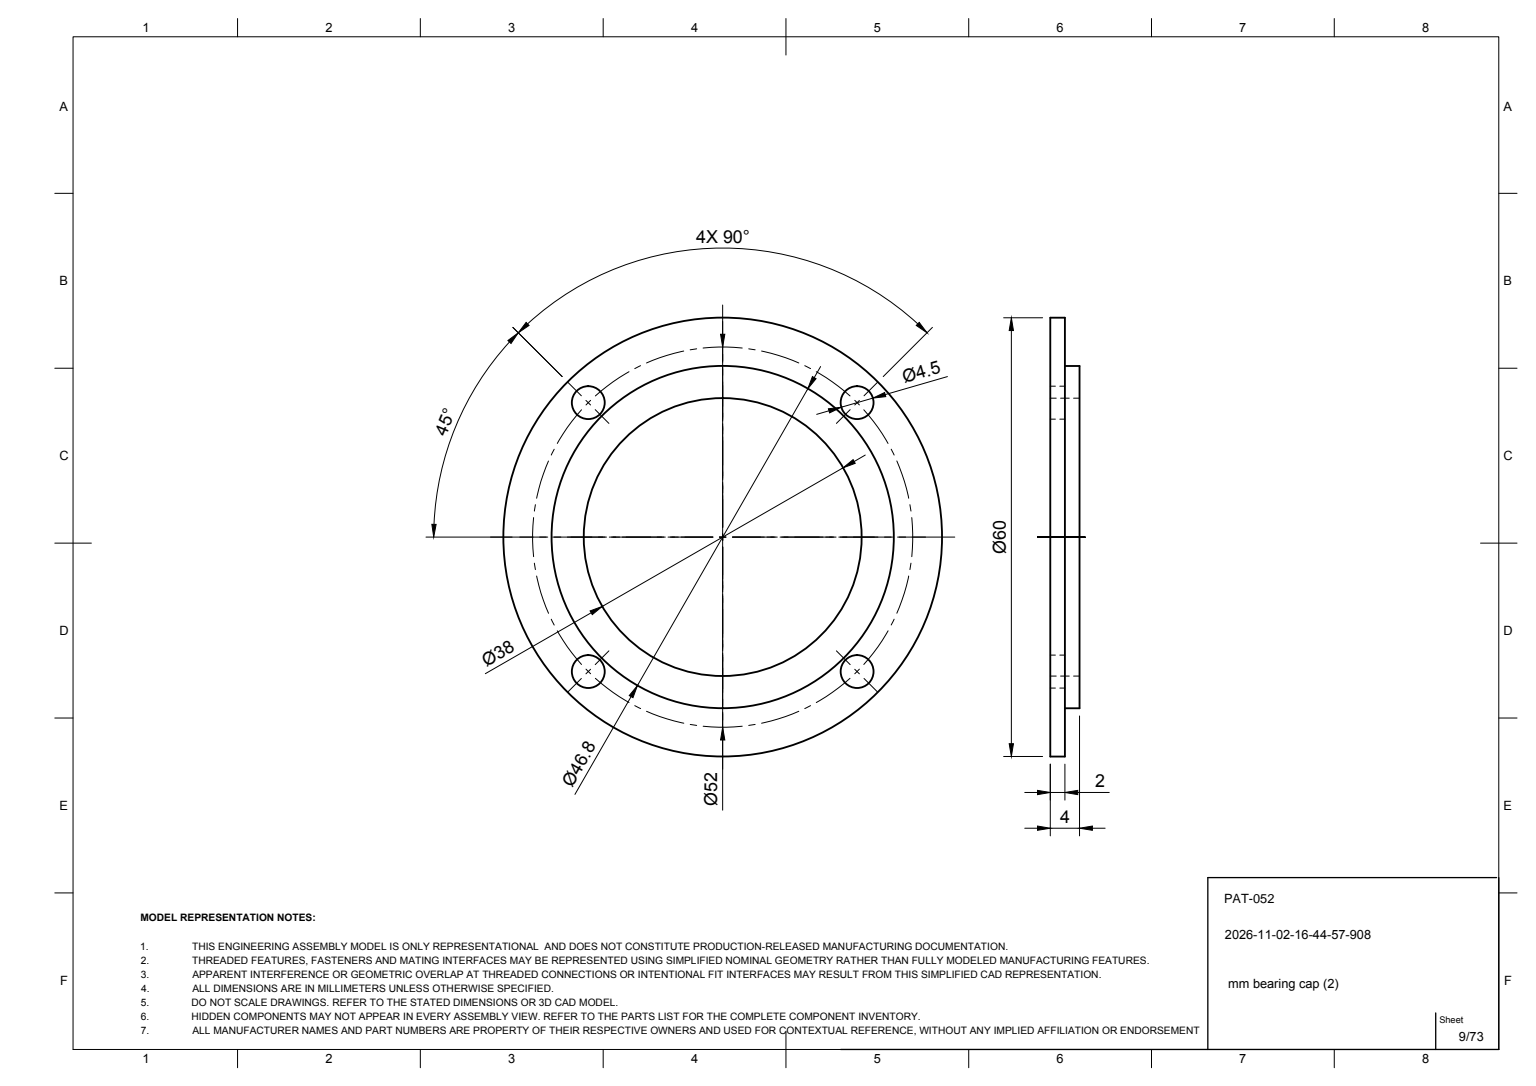
ISO-10303-21;
HEADER;
/* Generated by software containing ST-Developer
 * from STEP Tools, Inc. (www.steptools.com) 
 */

FILE_DESCRIPTION(
/* description */ ('Hand-crank gear train demonstrator'),
/* implementation_level */ '2;1');

FILE_NAME(
/* name */ 'mm bearing cap (2).step',
/* time_stamp */ '2026-10-28T03:22:13-07:00',
/* author */ (''),
/* organization */ (''),
/* preprocessor_version */ 'ST-DEVELOPER v20.2',
/* originating_system */ 'Autodesk Translation Framework v15.17.0.0',
/* authorisation */ '');

FILE_SCHEMA (('AUTOMOTIVE_DESIGN { 1 0 10303 214 3 1 1 }'));
ENDSEC;

DATA;
#10=MECHANICAL_DESIGN_GEOMETRIC_PRESENTATION_REPRESENTATION('',(#1193),#62758);
#1065=SHAPE_REPRESENTATION_RELATIONSHIP('SRR','None',#63037,#1129);
#1129=ADVANCED_BREP_SHAPE_REPRESENTATION('',(#1272),#62691);
#1193=STYLED_ITEM('',(#63462),#1272);
#1272=MANIFOLD_SOLID_BREP('Body1',#16373);
#1420=FACE_BOUND('',#3205,.T.);
#1421=FACE_BOUND('',#3209,.T.);
#1422=FACE_BOUND('',#3210,.T.);
#1423=FACE_BOUND('',#3211,.T.);
#1424=FACE_BOUND('',#3212,.T.);
#1425=FACE_BOUND('',#3213,.T.);
#1426=FACE_BOUND('',#3215,.T.);
#1427=FACE_BOUND('',#3216,.T.);
#1428=FACE_BOUND('',#3217,.T.);
#1429=FACE_BOUND('',#3218,.T.);
#1430=FACE_BOUND('',#3219,.T.);
#1653=PLANE('',#17326);
#1654=PLANE('',#17333);
#1655=PLANE('',#17334);
#2185=FACE_OUTER_BOUND('',#3199,.T.);
#2186=FACE_OUTER_BOUND('',#3200,.T.);
#2187=FACE_OUTER_BOUND('',#3201,.T.);
#2188=FACE_OUTER_BOUND('',#3202,.T.);
#2189=FACE_OUTER_BOUND('',#3203,.T.);
#2190=FACE_OUTER_BOUND('',#3204,.T.);
#2191=FACE_OUTER_BOUND('',#3206,.T.);
#2192=FACE_OUTER_BOUND('',#3207,.T.);
#2193=FACE_OUTER_BOUND('',#3208,.T.);
#2194=FACE_OUTER_BOUND('',#3214,.T.);
#3199=EDGE_LOOP('',(#11147,#11148,#11149,#11150));
#3200=EDGE_LOOP('',(#11151,#11152,#11153,#11154));
#3201=EDGE_LOOP('',(#11155,#11156,#11157,#11158));
#3202=EDGE_LOOP('',(#11159,#11160,#11161,#11162));
#3203=EDGE_LOOP('',(#11163,#11164,#11165,#11166));
#3204=EDGE_LOOP('',(#11167));
#3205=EDGE_LOOP('',(#11168));
#3206=EDGE_LOOP('',(#11169,#11170,#11171,#11172));
#3207=EDGE_LOOP('',(#11173,#11174,#11175,#11176));
#3208=EDGE_LOOP('',(#11177));
#3209=EDGE_LOOP('',(#11178));
#3210=EDGE_LOOP('',(#11179));
#3211=EDGE_LOOP('',(#11180));
#3212=EDGE_LOOP('',(#11181));
#3213=EDGE_LOOP('',(#11182));
#3214=EDGE_LOOP('',(#11183));
#3215=EDGE_LOOP('',(#11184));
#3216=EDGE_LOOP('',(#11185));
#3217=EDGE_LOOP('',(#11186));
#3218=EDGE_LOOP('',(#11187));
#3219=EDGE_LOOP('',(#11188));
#4358=LINE('',#23642,#5490);
#4359=LINE('',#23648,#5491);
#4360=LINE('',#23654,#5492);
#4361=LINE('',#23660,#5493);
#4362=LINE('',#23666,#5494);
#4363=LINE('',#23673,#5495);
#4364=LINE('',#23679,#5496);
#5490=VECTOR('',#19213,0.225);
#5491=VECTOR('',#19220,0.225);
#5492=VECTOR('',#19227,0.225000000000001);
#5493=VECTOR('',#19234,0.225000000000001);
#5494=VECTOR('',#19241,2.34);
#5495=VECTOR('',#19250,1.9);
#5496=VECTOR('',#19257,3.);
#6634=CIRCLE('',#17312,0.225);
#6635=CIRCLE('',#17313,0.225);
#6636=CIRCLE('',#17315,0.225);
#6637=CIRCLE('',#17316,0.225);
#6638=CIRCLE('',#17318,0.225000000000001);
#6639=CIRCLE('',#17319,0.225000000000001);
#6640=CIRCLE('',#17321,0.225000000000001);
#6641=CIRCLE('',#17322,0.225000000000001);
#6642=CIRCLE('',#17324,2.34);
#6643=CIRCLE('',#17325,2.34);
#6644=CIRCLE('',#17327,1.9);
#6645=CIRCLE('',#17329,1.9);
#6646=CIRCLE('',#17331,3.);
#6647=CIRCLE('',#17332,3.);
#7316=VERTEX_POINT('',#23639);
#7317=VERTEX_POINT('',#23641);
#7318=VERTEX_POINT('',#23645);
#7319=VERTEX_POINT('',#23647);
#7320=VERTEX_POINT('',#23651);
#7321=VERTEX_POINT('',#23653);
#7322=VERTEX_POINT('',#23657);
#7323=VERTEX_POINT('',#23659);
#7324=VERTEX_POINT('',#23663);
#7325=VERTEX_POINT('',#23665);
#7326=VERTEX_POINT('',#23669);
#7327=VERTEX_POINT('',#23672);
#7328=VERTEX_POINT('',#23676);
#7329=VERTEX_POINT('',#23678);
#8825=EDGE_CURVE('',#7316,#7316,#6634,.T.);
#8826=EDGE_CURVE('',#7316,#7317,#4358,.T.);
#8827=EDGE_CURVE('',#7317,#7317,#6635,.T.);
#8828=EDGE_CURVE('',#7318,#7318,#6636,.T.);
#8829=EDGE_CURVE('',#7318,#7319,#4359,.T.);
#8830=EDGE_CURVE('',#7319,#7319,#6637,.T.);
#8831=EDGE_CURVE('',#7320,#7320,#6638,.T.);
#8832=EDGE_CURVE('',#7320,#7321,#4360,.T.);
#8833=EDGE_CURVE('',#7321,#7321,#6639,.T.);
#8834=EDGE_CURVE('',#7322,#7322,#6640,.T.);
#8835=EDGE_CURVE('',#7322,#7323,#4361,.T.);
#8836=EDGE_CURVE('',#7323,#7323,#6641,.T.);
#8837=EDGE_CURVE('',#7324,#7324,#6642,.T.);
#8838=EDGE_CURVE('',#7324,#7325,#4362,.T.);
#8839=EDGE_CURVE('',#7325,#7325,#6643,.T.);
#8840=EDGE_CURVE('',#7326,#7326,#6644,.T.);
#8841=EDGE_CURVE('',#7326,#7327,#4363,.T.);
#8842=EDGE_CURVE('',#7327,#7327,#6645,.T.);
#8843=EDGE_CURVE('',#7328,#7328,#6646,.T.);
#8844=EDGE_CURVE('',#7328,#7329,#4364,.T.);
#8845=EDGE_CURVE('',#7329,#7329,#6647,.T.);
#11147=ORIENTED_EDGE('',*,*,#8825,.F.);
#11148=ORIENTED_EDGE('',*,*,#8826,.T.);
#11149=ORIENTED_EDGE('',*,*,#8827,.F.);
#11150=ORIENTED_EDGE('',*,*,#8826,.F.);
#11151=ORIENTED_EDGE('',*,*,#8828,.F.);
#11152=ORIENTED_EDGE('',*,*,#8829,.T.);
#11153=ORIENTED_EDGE('',*,*,#8830,.F.);
#11154=ORIENTED_EDGE('',*,*,#8829,.F.);
#11155=ORIENTED_EDGE('',*,*,#8831,.F.);
#11156=ORIENTED_EDGE('',*,*,#8832,.T.);
#11157=ORIENTED_EDGE('',*,*,#8833,.F.);
#11158=ORIENTED_EDGE('',*,*,#8832,.F.);
#11159=ORIENTED_EDGE('',*,*,#8834,.F.);
#11160=ORIENTED_EDGE('',*,*,#8835,.T.);
#11161=ORIENTED_EDGE('',*,*,#8836,.F.);
#11162=ORIENTED_EDGE('',*,*,#8835,.F.);
#11163=ORIENTED_EDGE('',*,*,#8837,.F.);
#11164=ORIENTED_EDGE('',*,*,#8838,.T.);
#11165=ORIENTED_EDGE('',*,*,#8839,.F.);
#11166=ORIENTED_EDGE('',*,*,#8838,.F.);
#11167=ORIENTED_EDGE('',*,*,#8837,.T.);
#11168=ORIENTED_EDGE('',*,*,#8840,.T.);
#11169=ORIENTED_EDGE('',*,*,#8840,.F.);
#11170=ORIENTED_EDGE('',*,*,#8841,.T.);
#11171=ORIENTED_EDGE('',*,*,#8842,.T.);
#11172=ORIENTED_EDGE('',*,*,#8841,.F.);
#11173=ORIENTED_EDGE('',*,*,#8843,.F.);
#11174=ORIENTED_EDGE('',*,*,#8844,.T.);
#11175=ORIENTED_EDGE('',*,*,#8845,.T.);
#11176=ORIENTED_EDGE('',*,*,#8844,.F.);
#11177=ORIENTED_EDGE('',*,*,#8843,.T.);
#11178=ORIENTED_EDGE('',*,*,#8839,.T.);
#11179=ORIENTED_EDGE('',*,*,#8836,.T.);
#11180=ORIENTED_EDGE('',*,*,#8833,.T.);
#11181=ORIENTED_EDGE('',*,*,#8830,.T.);
#11182=ORIENTED_EDGE('',*,*,#8827,.T.);
#11183=ORIENTED_EDGE('',*,*,#8845,.F.);
#11184=ORIENTED_EDGE('',*,*,#8842,.F.);
#11185=ORIENTED_EDGE('',*,*,#8834,.T.);
#11186=ORIENTED_EDGE('',*,*,#8831,.T.);
#11187=ORIENTED_EDGE('',*,*,#8828,.T.);
#11188=ORIENTED_EDGE('',*,*,#8825,.T.);
#15209=CYLINDRICAL_SURFACE('',#17311,0.225);
#15210=CYLINDRICAL_SURFACE('',#17314,0.225);
#15211=CYLINDRICAL_SURFACE('',#17317,0.225000000000001);
#15212=CYLINDRICAL_SURFACE('',#17320,0.225000000000001);
#15213=CYLINDRICAL_SURFACE('',#17323,2.34);
#15214=CYLINDRICAL_SURFACE('',#17328,1.9);
#15215=CYLINDRICAL_SURFACE('',#17330,3.);
#15495=ADVANCED_FACE('',(#2185),#15209,.F.);
#15496=ADVANCED_FACE('',(#2186),#15210,.F.);
#15497=ADVANCED_FACE('',(#2187),#15211,.F.);
#15498=ADVANCED_FACE('',(#2188),#15212,.F.);
#15499=ADVANCED_FACE('',(#2189),#15213,.T.);
#15500=ADVANCED_FACE('',(#2190,#1420),#1653,.T.);
#15501=ADVANCED_FACE('',(#2191),#15214,.F.);
#15502=ADVANCED_FACE('',(#2192),#15215,.T.);
#15503=ADVANCED_FACE('',(#2193,#1421,#1422,#1423,#1424,#1425),#1654,.T.);
#15504=ADVANCED_FACE('',(#2194,#1426,#1427,#1428,#1429,#1430),#1655,.F.);
#16373=CLOSED_SHELL('',(#15495,#15496,#15497,#15498,#15499,#15500,#15501,
#15502,#15503,#15504));
#17310=AXIS2_PLACEMENT_3D('',#23637,#19207,#19208);
#17311=AXIS2_PLACEMENT_3D('',#23638,#19209,#19210);
#17312=AXIS2_PLACEMENT_3D('',#23640,#19211,#19212);
#17313=AXIS2_PLACEMENT_3D('',#23643,#19214,#19215);
#17314=AXIS2_PLACEMENT_3D('',#23644,#19216,#19217);
#17315=AXIS2_PLACEMENT_3D('',#23646,#19218,#19219);
#17316=AXIS2_PLACEMENT_3D('',#23649,#19221,#19222);
#17317=AXIS2_PLACEMENT_3D('',#23650,#19223,#19224);
#17318=AXIS2_PLACEMENT_3D('',#23652,#19225,#19226);
#17319=AXIS2_PLACEMENT_3D('',#23655,#19228,#19229);
#17320=AXIS2_PLACEMENT_3D('',#23656,#19230,#19231);
#17321=AXIS2_PLACEMENT_3D('',#23658,#19232,#19233);
#17322=AXIS2_PLACEMENT_3D('',#23661,#19235,#19236);
#17323=AXIS2_PLACEMENT_3D('',#23662,#19237,#19238);
#17324=AXIS2_PLACEMENT_3D('',#23664,#19239,#19240);
#17325=AXIS2_PLACEMENT_3D('',#23667,#19242,#19243);
#17326=AXIS2_PLACEMENT_3D('',#23668,#19244,#19245);
#17327=AXIS2_PLACEMENT_3D('',#23670,#19246,#19247);
#17328=AXIS2_PLACEMENT_3D('',#23671,#19248,#19249);
#17329=AXIS2_PLACEMENT_3D('',#23674,#19251,#19252);
#17330=AXIS2_PLACEMENT_3D('',#23675,#19253,#19254);
#17331=AXIS2_PLACEMENT_3D('',#23677,#19255,#19256);
#17332=AXIS2_PLACEMENT_3D('',#23680,#19258,#19259);
#17333=AXIS2_PLACEMENT_3D('',#23681,#19260,#19261);
#17334=AXIS2_PLACEMENT_3D('',#23682,#19262,#19263);
#19207=DIRECTION('axis',(0.,0.,1.));
#19208=DIRECTION('refdir',(1.,0.,0.));
#19209=DIRECTION('center_axis',(0.,1.,0.));
#19210=DIRECTION('ref_axis',(1.,0.,0.));
#19211=DIRECTION('center_axis',(0.,1.,0.));
#19212=DIRECTION('ref_axis',(1.,0.,0.));
#19213=DIRECTION('',(0.,1.,0.));
#19214=DIRECTION('center_axis',(0.,-1.,0.));
#19215=DIRECTION('ref_axis',(1.,0.,0.));
#19216=DIRECTION('center_axis',(0.,1.,0.));
#19217=DIRECTION('ref_axis',(1.,0.,0.));
#19218=DIRECTION('center_axis',(0.,1.,0.));
#19219=DIRECTION('ref_axis',(1.,0.,0.));
#19220=DIRECTION('',(0.,1.,0.));
#19221=DIRECTION('center_axis',(0.,-1.,0.));
#19222=DIRECTION('ref_axis',(1.,0.,0.));
#19223=DIRECTION('center_axis',(0.,1.,0.));
#19224=DIRECTION('ref_axis',(1.,0.,0.));
#19225=DIRECTION('center_axis',(0.,1.,0.));
#19226=DIRECTION('ref_axis',(1.,0.,0.));
#19227=DIRECTION('',(0.,1.,0.));
#19228=DIRECTION('center_axis',(0.,-1.,0.));
#19229=DIRECTION('ref_axis',(1.,0.,0.));
#19230=DIRECTION('center_axis',(0.,1.,0.));
#19231=DIRECTION('ref_axis',(1.,0.,0.));
#19232=DIRECTION('center_axis',(0.,1.,0.));
#19233=DIRECTION('ref_axis',(1.,0.,0.));
#19234=DIRECTION('',(0.,1.,0.));
#19235=DIRECTION('center_axis',(0.,-1.,0.));
#19236=DIRECTION('ref_axis',(1.,0.,0.));
#19237=DIRECTION('center_axis',(0.,1.,0.));
#19238=DIRECTION('ref_axis',(1.,0.,0.));
#19239=DIRECTION('center_axis',(0.,1.,0.));
#19240=DIRECTION('ref_axis',(1.,0.,0.));
#19241=DIRECTION('',(0.,-1.,0.));
#19242=DIRECTION('center_axis',(0.,-1.,0.));
#19243=DIRECTION('ref_axis',(1.,0.,0.));
#19244=DIRECTION('center_axis',(0.,1.,0.));
#19245=DIRECTION('ref_axis',(1.,0.,0.));
#19246=DIRECTION('center_axis',(0.,-1.,0.));
#19247=DIRECTION('ref_axis',(1.,0.,0.));
#19248=DIRECTION('center_axis',(0.,1.,0.));
#19249=DIRECTION('ref_axis',(1.,0.,0.));
#19250=DIRECTION('',(0.,-1.,0.));
#19251=DIRECTION('center_axis',(0.,-1.,0.));
#19252=DIRECTION('ref_axis',(1.,0.,0.));
#19253=DIRECTION('center_axis',(0.,1.,0.));
#19254=DIRECTION('ref_axis',(1.,0.,0.));
#19255=DIRECTION('center_axis',(0.,1.,0.));
#19256=DIRECTION('ref_axis',(1.,0.,0.));
#19257=DIRECTION('',(0.,-1.,0.));
#19258=DIRECTION('center_axis',(0.,1.,0.));
#19259=DIRECTION('ref_axis',(1.,0.,0.));
#19260=DIRECTION('center_axis',(0.,1.,0.));
#19261=DIRECTION('ref_axis',(1.,0.,0.));
#19262=DIRECTION('center_axis',(0.,1.,0.));
#19263=DIRECTION('ref_axis',(1.,0.,0.));
#23637=CARTESIAN_POINT('',(0.,0.,0.));
#23638=CARTESIAN_POINT('Origin',(4.16152236891498,-2.7,7.16152236891498));
#23639=CARTESIAN_POINT('',(3.93652236891498,-2.6,7.16152236891498));
#23640=CARTESIAN_POINT('Origin',(4.16152236891498,-2.6,7.16152236891498));
#23641=CARTESIAN_POINT('',(3.93652236891498,-2.4,7.16152236891498));
#23642=CARTESIAN_POINT('',(3.93652236891498,-2.7,7.16152236891498));
#23643=CARTESIAN_POINT('Origin',(4.16152236891498,-2.4,7.16152236891498));
#23644=CARTESIAN_POINT('Origin',(4.16152236891498,-2.7,10.838477631085));
#23645=CARTESIAN_POINT('',(3.93652236891498,-2.6,10.838477631085));
#23646=CARTESIAN_POINT('Origin',(4.16152236891498,-2.6,10.838477631085));
#23647=CARTESIAN_POINT('',(3.93652236891498,-2.4,10.838477631085));
#23648=CARTESIAN_POINT('',(3.93652236891498,-2.7,10.838477631085));
#23649=CARTESIAN_POINT('Origin',(4.16152236891498,-2.4,10.838477631085));
#23650=CARTESIAN_POINT('Origin',(7.83847763108502,-2.7,10.838477631085));
#23651=CARTESIAN_POINT('',(7.61347763108502,-2.6,10.838477631085));
#23652=CARTESIAN_POINT('Origin',(7.83847763108502,-2.6,10.838477631085));
#23653=CARTESIAN_POINT('',(7.61347763108502,-2.4,10.838477631085));
#23654=CARTESIAN_POINT('',(7.61347763108502,-2.7,10.838477631085));
#23655=CARTESIAN_POINT('Origin',(7.83847763108502,-2.4,10.838477631085));
#23656=CARTESIAN_POINT('Origin',(7.83847763108502,-2.7,7.16152236891498));
#23657=CARTESIAN_POINT('',(7.61347763108502,-2.6,7.16152236891498));
#23658=CARTESIAN_POINT('Origin',(7.83847763108502,-2.6,7.16152236891498));
#23659=CARTESIAN_POINT('',(7.61347763108502,-2.4,7.16152236891498));
#23660=CARTESIAN_POINT('',(7.61347763108502,-2.7,7.16152236891498));
#23661=CARTESIAN_POINT('Origin',(7.83847763108502,-2.4,7.16152236891498));
#23662=CARTESIAN_POINT('Origin',(6.,-2.4,9.));
#23663=CARTESIAN_POINT('',(3.66,-2.2,9.));
#23664=CARTESIAN_POINT('Origin',(6.,-2.2,9.));
#23665=CARTESIAN_POINT('',(3.66,-2.4,9.));
#23666=CARTESIAN_POINT('',(3.66,-2.4,9.));
#23667=CARTESIAN_POINT('Origin',(6.,-2.4,9.));
#23668=CARTESIAN_POINT('Origin',(6.,-2.2,9.));
#23669=CARTESIAN_POINT('',(4.1,-2.2,9.));
#23670=CARTESIAN_POINT('Origin',(6.,-2.2,9.));
#23671=CARTESIAN_POINT('Origin',(6.,-2.6,9.));
#23672=CARTESIAN_POINT('',(4.1,-2.6,9.));
#23673=CARTESIAN_POINT('',(4.1,-2.6,9.));
#23674=CARTESIAN_POINT('Origin',(6.,-2.6,9.));
#23675=CARTESIAN_POINT('Origin',(6.,-2.6,9.));
#23676=CARTESIAN_POINT('',(3.,-2.4,9.));
#23677=CARTESIAN_POINT('Origin',(6.,-2.4,9.));
#23678=CARTESIAN_POINT('',(3.,-2.6,9.));
#23679=CARTESIAN_POINT('',(3.,-2.6,9.));
#23680=CARTESIAN_POINT('Origin',(6.,-2.6,9.));
#23681=CARTESIAN_POINT('Origin',(6.,-2.4,9.));
#23682=CARTESIAN_POINT('Origin',(6.,-2.6,9.));
#62617=UNCERTAINTY_MEASURE_WITH_UNIT(LENGTH_MEASURE(0.001),#62759,
'DISTANCE_ACCURACY_VALUE',
'Maximum model space distance between geometric entities at asserted c
onnectivities');
#62684=UNCERTAINTY_MEASURE_WITH_UNIT(LENGTH_MEASURE(0.001),#62759,
'DISTANCE_ACCURACY_VALUE',
'Maximum model space distance between geometric entities at asserted c
onnectivities');
#62691=(
GEOMETRIC_REPRESENTATION_CONTEXT(3)
GLOBAL_UNCERTAINTY_ASSIGNED_CONTEXT((#62617))
GLOBAL_UNIT_ASSIGNED_CONTEXT((#62759,#62761,#62762))
REPRESENTATION_CONTEXT('','3D')
);
#62758=(
GEOMETRIC_REPRESENTATION_CONTEXT(3)
GLOBAL_UNCERTAINTY_ASSIGNED_CONTEXT((#62684))
GLOBAL_UNIT_ASSIGNED_CONTEXT((#62759,#62761,#62762))
REPRESENTATION_CONTEXT('','3D')
);
#62759=(
LENGTH_UNIT()
NAMED_UNIT(*)
SI_UNIT(.CENTI.,.METRE.)
);
#62761=(
NAMED_UNIT(*)
PLANE_ANGLE_UNIT()
SI_UNIT($,.RADIAN.)
);
#62762=(
NAMED_UNIT(*)
SI_UNIT($,.STERADIAN.)
SOLID_ANGLE_UNIT()
);
#62769=SHAPE_DEFINITION_REPRESENTATION(#62842,#63037);
#62842=PRODUCT_DEFINITION_SHAPE('',$,#63111);
#63037=SHAPE_REPRESENTATION('',(#17310),#62691);
#63104=PRODUCT_DEFINITION_CONTEXT('part definition',#63325,'design');
#63111=PRODUCT_DEFINITION('mm bearing cap (2)','mm bearing cap (2)',#63184,
#63104);
#63184=PRODUCT_DEFINITION_FORMATION('',$,#63333);
#63325=APPLICATION_CONTEXT(
'Core Data for Automotive Mechanical Design Process');
#63326=PRODUCT_CONTEXT('part definition',#63325,'mechanical');
#63333=PRODUCT('mm bearing cap (2)','mm bearing cap (2)','mm bearing cap (2)',
(#63326));
#63456=COLOUR_RGB('Grey',0.48,0.52,0.57);
#63457=FILL_AREA_STYLE_COLOUR('',#63456);
#63458=FILL_AREA_STYLE('',(#63457));
#63459=SURFACE_STYLE_FILL_AREA(#63458);
#63460=SURFACE_SIDE_STYLE('',(#63459));
#63461=SURFACE_STYLE_USAGE(.BOTH.,#63460);
#63462=PRESENTATION_STYLE_ASSIGNMENT((#63461));
ENDSEC;
END-ISO-10303-21;
